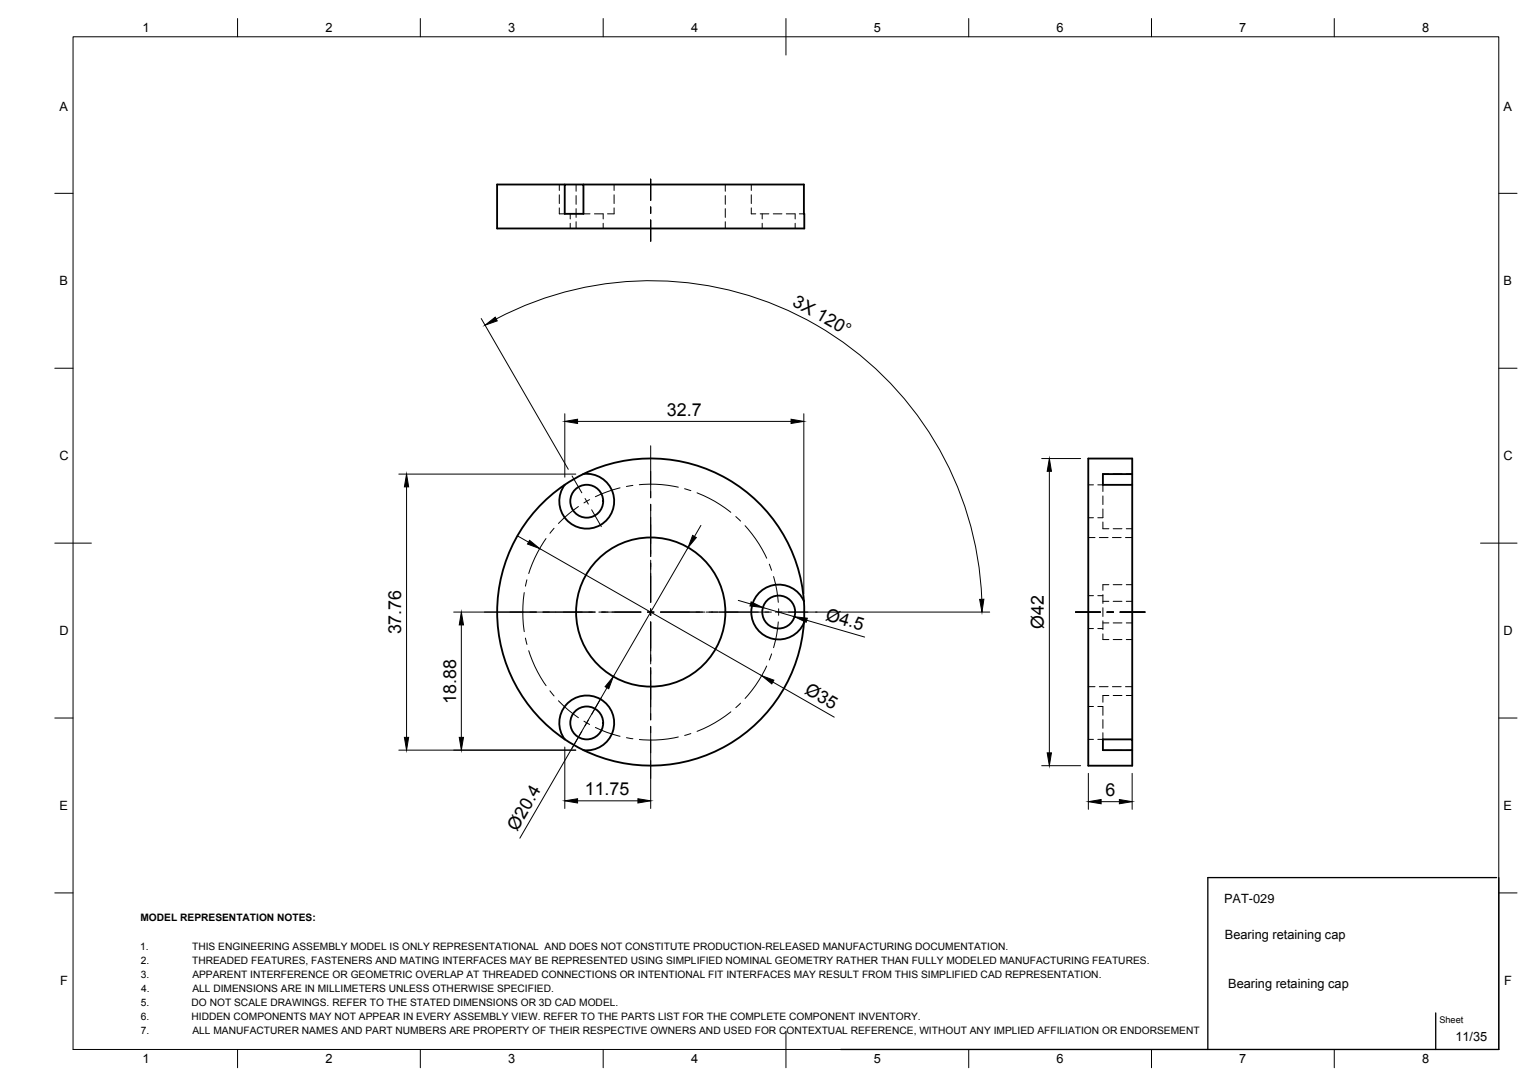
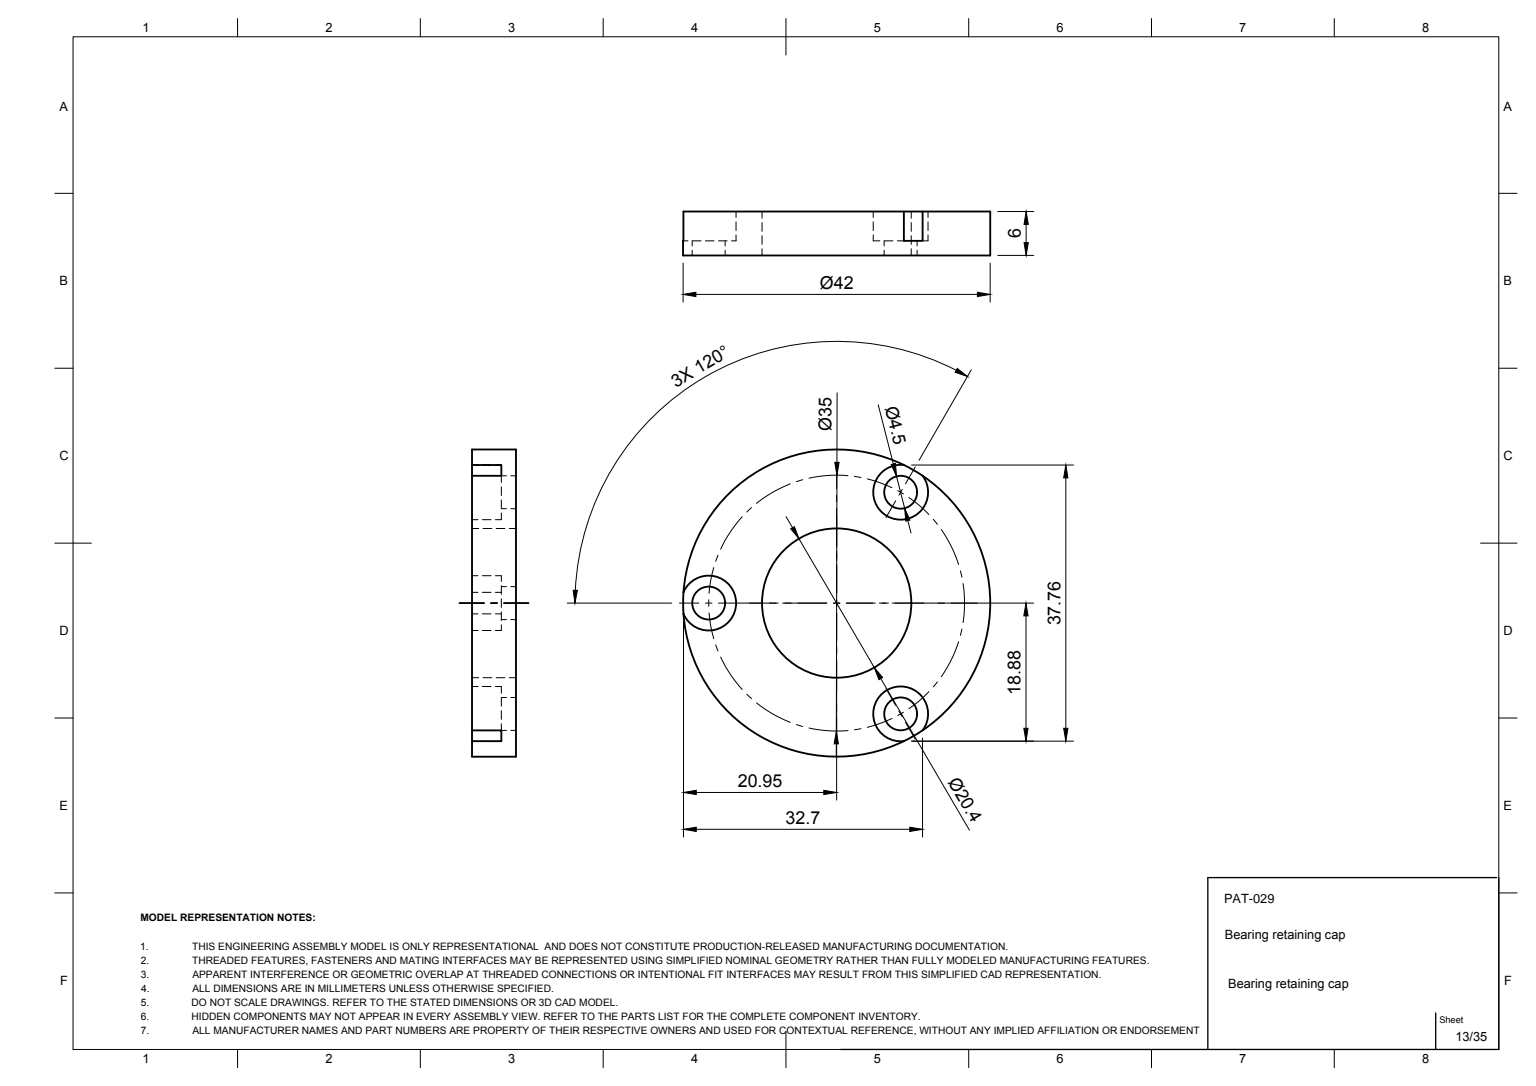
ISO-10303-21;
HEADER;
/* Generated by software containing ST-Developer
 * from STEP Tools, Inc. (www.steptools.com) 
 */

FILE_DESCRIPTION(
/* description */ ('Door-style hinge test fixture with detent'),
/* implementation_level */ '2;1');

FILE_NAME(
/* name */ 'Bearing retaining cap.step',
/* time_stamp */ '2026-10-28T03:24:57-07:00',
/* author */ (''),
/* organization */ (''),
/* preprocessor_version */ 'ST-DEVELOPER v20.2',
/* originating_system */ 'Autodesk Translation Framework v15.17.0.0',
/* authorisation */ '');

FILE_SCHEMA (('AUTOMOTIVE_DESIGN { 1 0 10303 214 3 1 1 }'));
ENDSEC;

DATA;
#10=MECHANICAL_DESIGN_GEOMETRIC_PRESENTATION_REPRESENTATION('',(#329),#9813);
#266=SHAPE_REPRESENTATION_RELATIONSHIP('SRR','None',#9943,#297);
#297=ADVANCED_BREP_SHAPE_REPRESENTATION('',(#369),#9786);
#329=STYLED_ITEM('',(#10183),#369);
#369=MANIFOLD_SOLID_BREP('Body1',#4760);
#432=FACE_BOUND('',#1042,.T.);
#433=FACE_BOUND('',#1045,.T.);
#434=FACE_BOUND('',#1048,.T.);
#435=FACE_BOUND('',#1056,.T.);
#436=FACE_BOUND('',#1058,.T.);
#437=FACE_BOUND('',#1059,.T.);
#438=FACE_BOUND('',#1060,.T.);
#439=FACE_BOUND('',#1061,.T.);
#542=PLANE('',#5243);
#543=PLANE('',#5249);
#544=PLANE('',#5255);
#545=PLANE('',#5276);
#546=PLANE('',#5277);
#723=FACE_OUTER_BOUND('',#1041,.T.);
#724=FACE_OUTER_BOUND('',#1043,.T.);
#725=FACE_OUTER_BOUND('',#1044,.T.);
#726=FACE_OUTER_BOUND('',#1046,.T.);
#727=FACE_OUTER_BOUND('',#1047,.T.);
#728=FACE_OUTER_BOUND('',#1049,.T.);
#729=FACE_OUTER_BOUND('',#1050,.T.);
#730=FACE_OUTER_BOUND('',#1051,.T.);
#731=FACE_OUTER_BOUND('',#1052,.T.);
#732=FACE_OUTER_BOUND('',#1053,.T.);
#733=FACE_OUTER_BOUND('',#1054,.T.);
#734=FACE_OUTER_BOUND('',#1055,.T.);
#735=FACE_OUTER_BOUND('',#1057,.T.);
#1041=EDGE_LOOP('',(#3477,#3478));
#1042=EDGE_LOOP('',(#3479));
#1043=EDGE_LOOP('',(#3480,#3481,#3482,#3483));
#1044=EDGE_LOOP('',(#3484,#3485));
#1045=EDGE_LOOP('',(#3486));
#1046=EDGE_LOOP('',(#3487,#3488,#3489,#3490));
#1047=EDGE_LOOP('',(#3491,#3492));
#1048=EDGE_LOOP('',(#3493));
#1049=EDGE_LOOP('',(#3494,#3495,#3496,#3497));
#1050=EDGE_LOOP('',(#3498,#3499,#3500,#3501,#3502,#3503,#3504,#3505,#3506,
#3507,#3508,#3509,#3510,#3511,#3512,#3513));
#1051=EDGE_LOOP('',(#3514,#3515,#3516,#3517));
#1052=EDGE_LOOP('',(#3518,#3519,#3520,#3521));
#1053=EDGE_LOOP('',(#3522,#3523,#3524,#3525));
#1054=EDGE_LOOP('',(#3526,#3527,#3528,#3529));
#1055=EDGE_LOOP('',(#3530,#3531,#3532,#3533,#3534,#3535,#3536));
#1056=EDGE_LOOP('',(#3537));
#1057=EDGE_LOOP('',(#3538));
#1058=EDGE_LOOP('',(#3539));
#1059=EDGE_LOOP('',(#3540));
#1060=EDGE_LOOP('',(#3541));
#1061=EDGE_LOOP('',(#3542));
#1433=LINE('',#7600,#1753);
#1434=LINE('',#7603,#1754);
#1435=LINE('',#7613,#1755);
#1436=LINE('',#7616,#1756);
#1437=LINE('',#7626,#1757);
#1438=LINE('',#7629,#1758);
#1439=LINE('',#7635,#1759);
#1440=LINE('',#7642,#1760);
#1441=LINE('',#7646,#1761);
#1442=LINE('',#7650,#1762);
#1443=LINE('',#7655,#1763);
#1753=VECTOR('',#6070,1.);
#1754=VECTOR('',#6073,1.);
#1755=VECTOR('',#6084,1.);
#1756=VECTOR('',#6087,1.);
#1757=VECTOR('',#6098,1.);
#1758=VECTOR('',#6101,1.);
#1759=VECTOR('',#6108,2.1);
#1760=VECTOR('',#6119,0.225);
#1761=VECTOR('',#6124,0.225);
#1762=VECTOR('',#6129,0.225);
#1763=VECTOR('',#6134,1.02);
#2010=CIRCLE('',#5244,2.1);
#2011=CIRCLE('',#5245,0.375);
#2012=CIRCLE('',#5246,0.225);
#2013=CIRCLE('',#5248,0.375);
#2014=CIRCLE('',#5250,2.1);
#2015=CIRCLE('',#5251,0.375);
#2016=CIRCLE('',#5252,0.225);
#2017=CIRCLE('',#5254,0.375);
#2018=CIRCLE('',#5256,2.1);
#2019=CIRCLE('',#5257,0.375);
#2020=CIRCLE('',#5258,0.225);
#2021=CIRCLE('',#5260,0.375);
#2022=CIRCLE('',#5262,2.1);
#2023=CIRCLE('',#5263,2.1);
#2024=CIRCLE('',#5264,2.1);
#2025=CIRCLE('',#5265,2.1);
#2026=CIRCLE('',#5266,2.1);
#2027=CIRCLE('',#5268,0.225);
#2028=CIRCLE('',#5270,0.225);
#2029=CIRCLE('',#5272,0.225);
#2030=CIRCLE('',#5274,1.02);
#2031=CIRCLE('',#5275,1.02);
#2311=VERTEX_POINT('',#7592);
#2312=VERTEX_POINT('',#7593);
#2313=VERTEX_POINT('',#7596);
#2314=VERTEX_POINT('',#7599);
#2315=VERTEX_POINT('',#7601);
#2316=VERTEX_POINT('',#7605);
#2317=VERTEX_POINT('',#7606);
#2318=VERTEX_POINT('',#7609);
#2319=VERTEX_POINT('',#7612);
#2320=VERTEX_POINT('',#7614);
#2321=VERTEX_POINT('',#7618);
#2322=VERTEX_POINT('',#7619);
#2323=VERTEX_POINT('',#7622);
#2324=VERTEX_POINT('',#7625);
#2325=VERTEX_POINT('',#7627);
#2326=VERTEX_POINT('',#7632);
#2327=VERTEX_POINT('',#7634);
#2328=VERTEX_POINT('',#7640);
#2329=VERTEX_POINT('',#7644);
#2330=VERTEX_POINT('',#7648);
#2331=VERTEX_POINT('',#7652);
#2332=VERTEX_POINT('',#7654);
#2755=EDGE_CURVE('',#2311,#2312,#2010,.T.);
#2756=EDGE_CURVE('',#2311,#2312,#2011,.T.);
#2757=EDGE_CURVE('',#2313,#2313,#2012,.T.);
#2758=EDGE_CURVE('',#2314,#2311,#1433,.T.);
#2759=EDGE_CURVE('',#2315,#2314,#2013,.T.);
#2760=EDGE_CURVE('',#2312,#2315,#1434,.T.);
#2761=EDGE_CURVE('',#2316,#2317,#2014,.T.);
#2762=EDGE_CURVE('',#2316,#2317,#2015,.T.);
#2763=EDGE_CURVE('',#2318,#2318,#2016,.T.);
#2764=EDGE_CURVE('',#2319,#2316,#1435,.T.);
#2765=EDGE_CURVE('',#2320,#2319,#2017,.T.);
#2766=EDGE_CURVE('',#2317,#2320,#1436,.T.);
#2767=EDGE_CURVE('',#2321,#2322,#2018,.T.);
#2768=EDGE_CURVE('',#2321,#2322,#2019,.T.);
#2769=EDGE_CURVE('',#2323,#2323,#2020,.T.);
#2770=EDGE_CURVE('',#2324,#2321,#1437,.T.);
#2771=EDGE_CURVE('',#2325,#2324,#2021,.T.);
#2772=EDGE_CURVE('',#2322,#2325,#1438,.T.);
#2773=EDGE_CURVE('',#2324,#2315,#2022,.T.);
#2774=EDGE_CURVE('',#2326,#2325,#2023,.T.);
#2775=EDGE_CURVE('',#2326,#2327,#1439,.T.);
#2776=EDGE_CURVE('',#2327,#2327,#2024,.T.);
#2777=EDGE_CURVE('',#2319,#2326,#2025,.T.);
#2778=EDGE_CURVE('',#2314,#2320,#2026,.T.);
#2779=EDGE_CURVE('',#2328,#2328,#2027,.T.);
#2780=EDGE_CURVE('',#2328,#2313,#1440,.T.);
#2781=EDGE_CURVE('',#2329,#2329,#2028,.T.);
#2782=EDGE_CURVE('',#2329,#2318,#1441,.T.);
#2783=EDGE_CURVE('',#2330,#2330,#2029,.T.);
#2784=EDGE_CURVE('',#2330,#2323,#1442,.T.);
#2785=EDGE_CURVE('',#2331,#2331,#2030,.T.);
#2786=EDGE_CURVE('',#2331,#2332,#1443,.T.);
#2787=EDGE_CURVE('',#2332,#2332,#2031,.T.);
#3477=ORIENTED_EDGE('',*,*,#2755,.F.);
#3478=ORIENTED_EDGE('',*,*,#2756,.T.);
#3479=ORIENTED_EDGE('',*,*,#2757,.F.);
#3480=ORIENTED_EDGE('',*,*,#2758,.F.);
#3481=ORIENTED_EDGE('',*,*,#2759,.F.);
#3482=ORIENTED_EDGE('',*,*,#2760,.F.);
#3483=ORIENTED_EDGE('',*,*,#2756,.F.);
#3484=ORIENTED_EDGE('',*,*,#2761,.F.);
#3485=ORIENTED_EDGE('',*,*,#2762,.T.);
#3486=ORIENTED_EDGE('',*,*,#2763,.F.);
#3487=ORIENTED_EDGE('',*,*,#2764,.F.);
#3488=ORIENTED_EDGE('',*,*,#2765,.F.);
#3489=ORIENTED_EDGE('',*,*,#2766,.F.);
#3490=ORIENTED_EDGE('',*,*,#2762,.F.);
#3491=ORIENTED_EDGE('',*,*,#2767,.F.);
#3492=ORIENTED_EDGE('',*,*,#2768,.T.);
#3493=ORIENTED_EDGE('',*,*,#2769,.F.);
#3494=ORIENTED_EDGE('',*,*,#2770,.F.);
#3495=ORIENTED_EDGE('',*,*,#2771,.F.);
#3496=ORIENTED_EDGE('',*,*,#2772,.F.);
#3497=ORIENTED_EDGE('',*,*,#2768,.F.);
#3498=ORIENTED_EDGE('',*,*,#2758,.T.);
#3499=ORIENTED_EDGE('',*,*,#2755,.T.);
#3500=ORIENTED_EDGE('',*,*,#2760,.T.);
#3501=ORIENTED_EDGE('',*,*,#2773,.F.);
#3502=ORIENTED_EDGE('',*,*,#2770,.T.);
#3503=ORIENTED_EDGE('',*,*,#2767,.T.);
#3504=ORIENTED_EDGE('',*,*,#2772,.T.);
#3505=ORIENTED_EDGE('',*,*,#2774,.F.);
#3506=ORIENTED_EDGE('',*,*,#2775,.T.);
#3507=ORIENTED_EDGE('',*,*,#2776,.T.);
#3508=ORIENTED_EDGE('',*,*,#2775,.F.);
#3509=ORIENTED_EDGE('',*,*,#2777,.F.);
#3510=ORIENTED_EDGE('',*,*,#2764,.T.);
#3511=ORIENTED_EDGE('',*,*,#2761,.T.);
#3512=ORIENTED_EDGE('',*,*,#2766,.T.);
#3513=ORIENTED_EDGE('',*,*,#2778,.F.);
#3514=ORIENTED_EDGE('',*,*,#2779,.F.);
#3515=ORIENTED_EDGE('',*,*,#2780,.T.);
#3516=ORIENTED_EDGE('',*,*,#2757,.T.);
#3517=ORIENTED_EDGE('',*,*,#2780,.F.);
#3518=ORIENTED_EDGE('',*,*,#2781,.F.);
#3519=ORIENTED_EDGE('',*,*,#2782,.T.);
#3520=ORIENTED_EDGE('',*,*,#2763,.T.);
#3521=ORIENTED_EDGE('',*,*,#2782,.F.);
#3522=ORIENTED_EDGE('',*,*,#2783,.F.);
#3523=ORIENTED_EDGE('',*,*,#2784,.T.);
#3524=ORIENTED_EDGE('',*,*,#2769,.T.);
#3525=ORIENTED_EDGE('',*,*,#2784,.F.);
#3526=ORIENTED_EDGE('',*,*,#2785,.F.);
#3527=ORIENTED_EDGE('',*,*,#2786,.T.);
#3528=ORIENTED_EDGE('',*,*,#2787,.T.);
#3529=ORIENTED_EDGE('',*,*,#2786,.F.);
#3530=ORIENTED_EDGE('',*,*,#2759,.T.);
#3531=ORIENTED_EDGE('',*,*,#2778,.T.);
#3532=ORIENTED_EDGE('',*,*,#2765,.T.);
#3533=ORIENTED_EDGE('',*,*,#2777,.T.);
#3534=ORIENTED_EDGE('',*,*,#2774,.T.);
#3535=ORIENTED_EDGE('',*,*,#2771,.T.);
#3536=ORIENTED_EDGE('',*,*,#2773,.T.);
#3537=ORIENTED_EDGE('',*,*,#2785,.T.);
#3538=ORIENTED_EDGE('',*,*,#2776,.F.);
#3539=ORIENTED_EDGE('',*,*,#2779,.T.);
#3540=ORIENTED_EDGE('',*,*,#2781,.T.);
#3541=ORIENTED_EDGE('',*,*,#2783,.T.);
#3542=ORIENTED_EDGE('',*,*,#2787,.F.);
#4399=CYLINDRICAL_SURFACE('',#5247,0.375);
#4400=CYLINDRICAL_SURFACE('',#5253,0.375);
#4401=CYLINDRICAL_SURFACE('',#5259,0.375);
#4402=CYLINDRICAL_SURFACE('',#5261,2.1);
#4403=CYLINDRICAL_SURFACE('',#5267,0.225);
#4404=CYLINDRICAL_SURFACE('',#5269,0.225);
#4405=CYLINDRICAL_SURFACE('',#5271,0.225);
#4406=CYLINDRICAL_SURFACE('',#5273,1.02);
#4528=ADVANCED_FACE('',(#723,#432),#542,.T.);
#4529=ADVANCED_FACE('',(#724),#4399,.F.);
#4530=ADVANCED_FACE('',(#725,#433),#543,.T.);
#4531=ADVANCED_FACE('',(#726),#4400,.F.);
#4532=ADVANCED_FACE('',(#727,#434),#544,.T.);
#4533=ADVANCED_FACE('',(#728),#4401,.F.);
#4534=ADVANCED_FACE('',(#729),#4402,.T.);
#4535=ADVANCED_FACE('',(#730),#4403,.F.);
#4536=ADVANCED_FACE('',(#731),#4404,.F.);
#4537=ADVANCED_FACE('',(#732),#4405,.F.);
#4538=ADVANCED_FACE('',(#733),#4406,.F.);
#4539=ADVANCED_FACE('',(#734,#435),#545,.T.);
#4540=ADVANCED_FACE('',(#735,#436,#437,#438,#439),#546,.F.);
#4760=CLOSED_SHELL('',(#4528,#4529,#4530,#4531,#4532,#4533,#4534,#4535,
#4536,#4537,#4538,#4539,#4540));
#5242=AXIS2_PLACEMENT_3D('',#7590,#6058,#6059);
#5243=AXIS2_PLACEMENT_3D('',#7591,#6060,#6061);
#5244=AXIS2_PLACEMENT_3D('',#7594,#6062,#6063);
#5245=AXIS2_PLACEMENT_3D('',#7595,#6064,#6065);
#5246=AXIS2_PLACEMENT_3D('',#7597,#6066,#6067);
#5247=AXIS2_PLACEMENT_3D('',#7598,#6068,#6069);
#5248=AXIS2_PLACEMENT_3D('',#7602,#6071,#6072);
#5249=AXIS2_PLACEMENT_3D('',#7604,#6074,#6075);
#5250=AXIS2_PLACEMENT_3D('',#7607,#6076,#6077);
#5251=AXIS2_PLACEMENT_3D('',#7608,#6078,#6079);
#5252=AXIS2_PLACEMENT_3D('',#7610,#6080,#6081);
#5253=AXIS2_PLACEMENT_3D('',#7611,#6082,#6083);
#5254=AXIS2_PLACEMENT_3D('',#7615,#6085,#6086);
#5255=AXIS2_PLACEMENT_3D('',#7617,#6088,#6089);
#5256=AXIS2_PLACEMENT_3D('',#7620,#6090,#6091);
#5257=AXIS2_PLACEMENT_3D('',#7621,#6092,#6093);
#5258=AXIS2_PLACEMENT_3D('',#7623,#6094,#6095);
#5259=AXIS2_PLACEMENT_3D('',#7624,#6096,#6097);
#5260=AXIS2_PLACEMENT_3D('',#7628,#6099,#6100);
#5261=AXIS2_PLACEMENT_3D('',#7630,#6102,#6103);
#5262=AXIS2_PLACEMENT_3D('',#7631,#6104,#6105);
#5263=AXIS2_PLACEMENT_3D('',#7633,#6106,#6107);
#5264=AXIS2_PLACEMENT_3D('',#7636,#6109,#6110);
#5265=AXIS2_PLACEMENT_3D('',#7637,#6111,#6112);
#5266=AXIS2_PLACEMENT_3D('',#7638,#6113,#6114);
#5267=AXIS2_PLACEMENT_3D('',#7639,#6115,#6116);
#5268=AXIS2_PLACEMENT_3D('',#7641,#6117,#6118);
#5269=AXIS2_PLACEMENT_3D('',#7643,#6120,#6121);
#5270=AXIS2_PLACEMENT_3D('',#7645,#6122,#6123);
#5271=AXIS2_PLACEMENT_3D('',#7647,#6125,#6126);
#5272=AXIS2_PLACEMENT_3D('',#7649,#6127,#6128);
#5273=AXIS2_PLACEMENT_3D('',#7651,#6130,#6131);
#5274=AXIS2_PLACEMENT_3D('',#7653,#6132,#6133);
#5275=AXIS2_PLACEMENT_3D('',#7656,#6135,#6136);
#5276=AXIS2_PLACEMENT_3D('',#7657,#6137,#6138);
#5277=AXIS2_PLACEMENT_3D('',#7658,#6139,#6140);
#6058=DIRECTION('axis',(0.,0.,1.));
#6059=DIRECTION('refdir',(1.,0.,0.));
#6060=DIRECTION('center_axis',(0.,0.,1.));
#6061=DIRECTION('ref_axis',(1.,0.,0.));
#6062=DIRECTION('center_axis',(0.,0.,-1.));
#6063=DIRECTION('ref_axis',(1.,0.,0.));
#6064=DIRECTION('center_axis',(0.,0.,1.));
#6065=DIRECTION('ref_axis',(1.,0.,0.));
#6066=DIRECTION('center_axis',(0.,0.,1.));
#6067=DIRECTION('ref_axis',(1.,0.,0.));
#6068=DIRECTION('center_axis',(0.,0.,1.));
#6069=DIRECTION('ref_axis',(-1.,1.22464679914735E-16,0.));
#6070=DIRECTION('',(0.,0.,-1.));
#6071=DIRECTION('center_axis',(0.,0.,-1.));
#6072=DIRECTION('ref_axis',(1.,0.,0.));
#6073=DIRECTION('',(0.,0.,1.));
#6074=DIRECTION('center_axis',(0.,0.,1.));
#6075=DIRECTION('ref_axis',(1.,0.,0.));
#6076=DIRECTION('center_axis',(0.,0.,-1.));
#6077=DIRECTION('ref_axis',(1.,0.,0.));
#6078=DIRECTION('center_axis',(0.,0.,1.));
#6079=DIRECTION('ref_axis',(1.,0.,0.));
#6080=DIRECTION('center_axis',(0.,0.,1.));
#6081=DIRECTION('ref_axis',(1.,0.,0.));
#6082=DIRECTION('center_axis',(0.,0.,1.));
#6083=DIRECTION('ref_axis',(0.499999999999999,-0.866025403784439,0.));
#6084=DIRECTION('',(0.,0.,-1.));
#6085=DIRECTION('center_axis',(0.,0.,-1.));
#6086=DIRECTION('ref_axis',(1.,0.,0.));
#6087=DIRECTION('',(0.,0.,1.));
#6088=DIRECTION('center_axis',(0.,0.,1.));
#6089=DIRECTION('ref_axis',(1.,0.,0.));
#6090=DIRECTION('center_axis',(0.,0.,-1.));
#6091=DIRECTION('ref_axis',(1.,0.,0.));
#6092=DIRECTION('center_axis',(0.,0.,1.));
#6093=DIRECTION('ref_axis',(1.,0.,0.));
#6094=DIRECTION('center_axis',(0.,0.,1.));
#6095=DIRECTION('ref_axis',(1.,0.,0.));
#6096=DIRECTION('center_axis',(0.,0.,1.));
#6097=DIRECTION('ref_axis',(0.500000000000001,0.866025403784438,0.));
#6098=DIRECTION('',(0.,0.,-1.));
#6099=DIRECTION('center_axis',(0.,0.,-1.));
#6100=DIRECTION('ref_axis',(1.,0.,0.));
#6101=DIRECTION('',(0.,0.,1.));
#6102=DIRECTION('center_axis',(0.,0.,1.));
#6103=DIRECTION('ref_axis',(1.,0.,0.));
#6104=DIRECTION('center_axis',(0.,0.,1.));
#6105=DIRECTION('ref_axis',(1.,0.,0.));
#6106=DIRECTION('center_axis',(0.,0.,1.));
#6107=DIRECTION('ref_axis',(1.,0.,0.));
#6108=DIRECTION('',(0.,0.,-1.));
#6109=DIRECTION('center_axis',(0.,0.,1.));
#6110=DIRECTION('ref_axis',(1.,0.,0.));
#6111=DIRECTION('center_axis',(0.,0.,1.));
#6112=DIRECTION('ref_axis',(1.,0.,0.));
#6113=DIRECTION('center_axis',(0.,0.,1.));
#6114=DIRECTION('ref_axis',(1.,0.,0.));
#6115=DIRECTION('center_axis',(0.,0.,1.));
#6116=DIRECTION('ref_axis',(1.,0.,0.));
#6117=DIRECTION('center_axis',(0.,0.,1.));
#6118=DIRECTION('ref_axis',(1.,0.,0.));
#6119=DIRECTION('',(0.,0.,1.));
#6120=DIRECTION('center_axis',(0.,0.,1.));
#6121=DIRECTION('ref_axis',(1.,0.,0.));
#6122=DIRECTION('center_axis',(0.,0.,1.));
#6123=DIRECTION('ref_axis',(1.,0.,0.));
#6124=DIRECTION('',(0.,0.,1.));
#6125=DIRECTION('center_axis',(0.,0.,1.));
#6126=DIRECTION('ref_axis',(1.,0.,0.));
#6127=DIRECTION('center_axis',(0.,0.,1.));
#6128=DIRECTION('ref_axis',(1.,0.,0.));
#6129=DIRECTION('',(0.,0.,1.));
#6130=DIRECTION('center_axis',(0.,0.,1.));
#6131=DIRECTION('ref_axis',(1.,0.,0.));
#6132=DIRECTION('center_axis',(0.,0.,-1.));
#6133=DIRECTION('ref_axis',(1.,0.,0.));
#6134=DIRECTION('',(0.,0.,-1.));
#6135=DIRECTION('center_axis',(0.,0.,-1.));
#6136=DIRECTION('ref_axis',(1.,0.,0.));
#6137=DIRECTION('center_axis',(0.,0.,1.));
#6138=DIRECTION('ref_axis',(1.,0.,0.));
#6139=DIRECTION('center_axis',(0.,0.,1.));
#6140=DIRECTION('ref_axis',(1.,0.,0.));
#7590=CARTESIAN_POINT('',(0.,0.,0.));
#7591=CARTESIAN_POINT('Origin',(1.75,0.,3.6));
#7592=CARTESIAN_POINT('',(2.09482142857143,0.14738786380825,3.6));
#7593=CARTESIAN_POINT('',(2.09482142857143,-0.14738786380825,3.6));
#7594=CARTESIAN_POINT('Origin',(0.,0.,3.6));
#7595=CARTESIAN_POINT('Origin',(1.75,0.,3.6));
#7596=CARTESIAN_POINT('',(1.525,-2.75545529808155E-17,3.6));
#7597=CARTESIAN_POINT('Origin',(1.75,0.,3.6));
#7598=CARTESIAN_POINT('Origin',(1.75,0.,3.6));
#7599=CARTESIAN_POINT('',(2.09482142857143,0.147387863808251,4.));
#7600=CARTESIAN_POINT('',(2.09482142857143,0.14738786380825,3.6));
#7601=CARTESIAN_POINT('',(2.09482142857143,-0.147387863808251,4.));
#7602=CARTESIAN_POINT('Origin',(1.75,0.,4.));
#7603=CARTESIAN_POINT('',(2.09482142857143,-0.14738786380825,3.6));
#7604=CARTESIAN_POINT('Origin',(-0.875,1.51554445662277,3.6));
#7605=CARTESIAN_POINT('',(-1.17505234855318,1.74047464163074,3.6));
#7606=CARTESIAN_POINT('',(-0.919769080018249,1.88786250543899,3.6));
#7607=CARTESIAN_POINT('Origin',(0.,0.,3.6));
#7608=CARTESIAN_POINT('Origin',(-0.875,1.51554445662277,3.6));
#7609=CARTESIAN_POINT('',(-1.1,1.51554445662277,3.6));
#7610=CARTESIAN_POINT('Origin',(-0.875,1.51554445662277,3.6));
#7611=CARTESIAN_POINT('Origin',(-0.875,1.51554445662277,3.6));
#7612=CARTESIAN_POINT('',(-1.17505234855318,1.74047464163074,4.));
#7613=CARTESIAN_POINT('',(-1.17505234855318,1.74047464163074,3.6));
#7614=CARTESIAN_POINT('',(-0.919769080018247,1.88786250543899,4.));
#7615=CARTESIAN_POINT('Origin',(-0.875,1.51554445662277,4.));
#7616=CARTESIAN_POINT('',(-0.919769080018249,1.88786250543899,3.6));
#7617=CARTESIAN_POINT('Origin',(-0.875000000000001,-1.51554445662277,3.6));
#7618=CARTESIAN_POINT('',(-0.91976908001825,-1.88786250543899,3.6));
#7619=CARTESIAN_POINT('',(-1.17505234855318,-1.74047464163074,3.6));
#7620=CARTESIAN_POINT('Origin',(0.,0.,3.6));
#7621=CARTESIAN_POINT('Origin',(-0.875000000000001,-1.51554445662277,3.6));
#7622=CARTESIAN_POINT('',(-1.1,-1.51554445662277,3.6));
#7623=CARTESIAN_POINT('Origin',(-0.875000000000001,-1.51554445662277,3.6));
#7624=CARTESIAN_POINT('Origin',(-0.875000000000001,-1.51554445662277,3.6));
#7625=CARTESIAN_POINT('',(-0.919769080018249,-1.88786250543899,4.));
#7626=CARTESIAN_POINT('',(-0.91976908001825,-1.88786250543899,3.6));
#7627=CARTESIAN_POINT('',(-1.17505234855318,-1.74047464163074,4.));
#7628=CARTESIAN_POINT('Origin',(-0.875000000000001,-1.51554445662277,4.));
#7629=CARTESIAN_POINT('',(-1.17505234855318,-1.74047464163074,3.6));
#7630=CARTESIAN_POINT('Origin',(0.,0.,3.4));
#7631=CARTESIAN_POINT('Origin',(0.,0.,4.));
#7632=CARTESIAN_POINT('',(-2.1,-2.57175827820944E-16,4.));
#7633=CARTESIAN_POINT('Origin',(0.,0.,4.));
#7634=CARTESIAN_POINT('',(-2.1,-2.57175827820944E-16,3.4));
#7635=CARTESIAN_POINT('',(-2.1,-2.57175827820944E-16,3.4));
#7636=CARTESIAN_POINT('Origin',(0.,0.,3.4));
#7637=CARTESIAN_POINT('Origin',(0.,0.,4.));
#7638=CARTESIAN_POINT('Origin',(0.,0.,4.));
#7639=CARTESIAN_POINT('Origin',(1.75,0.,3.3));
#7640=CARTESIAN_POINT('',(1.525,-2.75545529808155E-17,3.4));
#7641=CARTESIAN_POINT('Origin',(1.75,0.,3.4));
#7642=CARTESIAN_POINT('',(1.525,-2.75545529808155E-17,3.3));
#7643=CARTESIAN_POINT('Origin',(-0.875,1.51554445662277,3.3));
#7644=CARTESIAN_POINT('',(-1.1,1.51554445662277,3.4));
#7645=CARTESIAN_POINT('Origin',(-0.875,1.51554445662277,3.4));
#7646=CARTESIAN_POINT('',(-1.1,1.51554445662277,3.3));
#7647=CARTESIAN_POINT('Origin',(-0.875000000000001,-1.51554445662277,3.3));
#7648=CARTESIAN_POINT('',(-1.1,-1.51554445662277,3.4));
#7649=CARTESIAN_POINT('Origin',(-0.875000000000001,-1.51554445662277,3.4));
#7650=CARTESIAN_POINT('',(-1.1,-1.51554445662277,3.3));
#7651=CARTESIAN_POINT('Origin',(0.,0.,3.4));
#7652=CARTESIAN_POINT('',(-1.02,-1.2491397351303E-16,4.));
#7653=CARTESIAN_POINT('Origin',(0.,0.,4.));
#7654=CARTESIAN_POINT('',(-1.02,-1.2491397351303E-16,3.4));
#7655=CARTESIAN_POINT('',(-1.02,-1.2491397351303E-16,3.4));
#7656=CARTESIAN_POINT('Origin',(0.,0.,3.4));
#7657=CARTESIAN_POINT('Origin',(0.,0.,4.));
#7658=CARTESIAN_POINT('Origin',(0.,0.,3.4));
#9750=UNCERTAINTY_MEASURE_WITH_UNIT(LENGTH_MEASURE(0.001),#9814,
'DISTANCE_ACCURACY_VALUE',
'Maximum model space distance between geometric entities at asserted c
onnectivities');
#9777=UNCERTAINTY_MEASURE_WITH_UNIT(LENGTH_MEASURE(0.001),#9814,
'DISTANCE_ACCURACY_VALUE',
'Maximum model space distance between geometric entities at asserted c
onnectivities');
#9786=(
GEOMETRIC_REPRESENTATION_CONTEXT(3)
GLOBAL_UNCERTAINTY_ASSIGNED_CONTEXT((#9750))
GLOBAL_UNIT_ASSIGNED_CONTEXT((#9814,#9816,#9817))
REPRESENTATION_CONTEXT('','3D')
);
#9813=(
GEOMETRIC_REPRESENTATION_CONTEXT(3)
GLOBAL_UNCERTAINTY_ASSIGNED_CONTEXT((#9777))
GLOBAL_UNIT_ASSIGNED_CONTEXT((#9814,#9816,#9817))
REPRESENTATION_CONTEXT('','3D')
);
#9814=(
LENGTH_UNIT()
NAMED_UNIT(*)
SI_UNIT(.CENTI.,.METRE.)
);
#9816=(
NAMED_UNIT(*)
PLANE_ANGLE_UNIT()
SI_UNIT($,.RADIAN.)
);
#9817=(
NAMED_UNIT(*)
SI_UNIT($,.STERADIAN.)
SOLID_ANGLE_UNIT()
);
#9826=SHAPE_DEFINITION_REPRESENTATION(#9861,#9943);
#9861=PRODUCT_DEFINITION_SHAPE('',$,#9979);
#9943=SHAPE_REPRESENTATION('',(#5242),#9786);
#9970=PRODUCT_DEFINITION_CONTEXT('part definition',#10077,'design');
#9979=PRODUCT_DEFINITION('Bearing retaining cap',
'Bearing retaining cap',#10014,#9970);
#10014=PRODUCT_DEFINITION_FORMATION('',$,#10087);
#10077=APPLICATION_CONTEXT(
'Core Data for Automotive Mechanical Design Process');
#10078=PRODUCT_CONTEXT('part definition',#10077,'mechanical');
#10087=PRODUCT('Bearing retaining cap','Bearing retaining cap',
'Bearing retaining cap',(#10078));
#10177=COLOUR_RGB('Grey',0.48,0.52,0.57);
#10178=FILL_AREA_STYLE_COLOUR('',#10177);
#10179=FILL_AREA_STYLE('',(#10178));
#10180=SURFACE_STYLE_FILL_AREA(#10179);
#10181=SURFACE_SIDE_STYLE('',(#10180));
#10182=SURFACE_STYLE_USAGE(.BOTH.,#10181);
#10183=PRESENTATION_STYLE_ASSIGNMENT((#10182));
ENDSEC;
END-ISO-10303-21;
